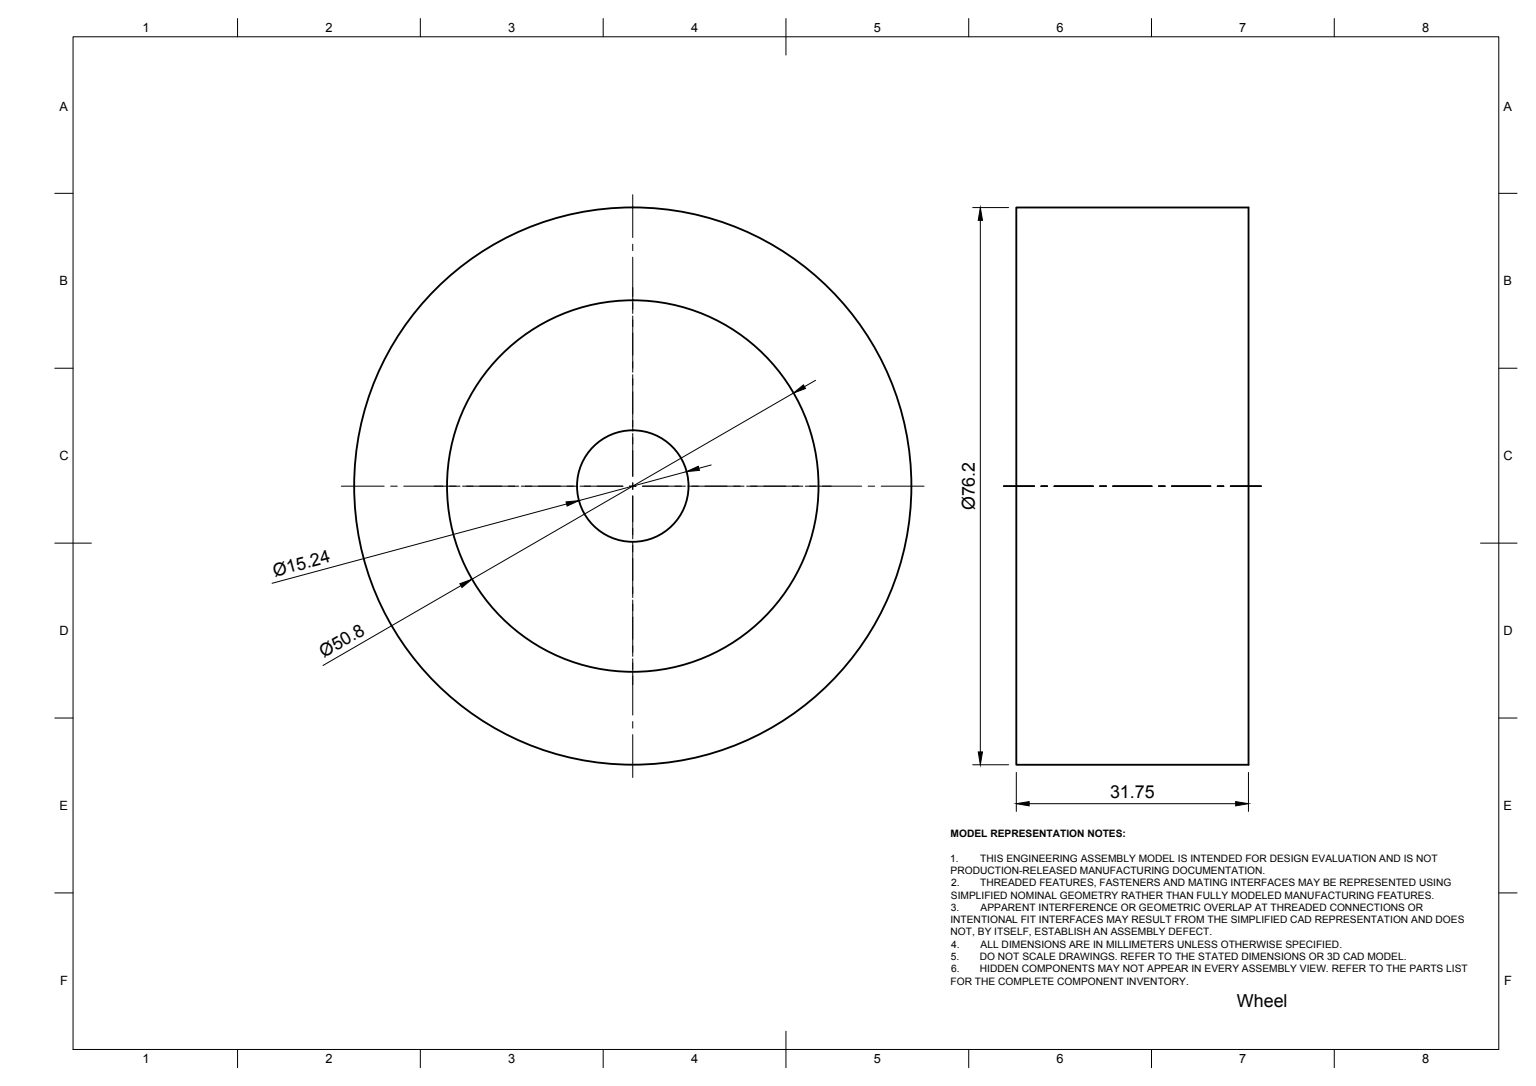
ISO-10303-21;
HEADER;
/* Generated by software containing ST-Developer
 * from STEP Tools, Inc. (www.steptools.com) 
 */

FILE_DESCRIPTION(
/* description */ ('Wheel Holder-Mirrored'),
/* implementation_level */ '2;1');

FILE_NAME(
/* name */ 'Wheel.step',
/* time_stamp */ '2026-10-07T09:01:46-07:00',
/* author */ (''),
/* organization */ (''),
/* preprocessor_version */ 'ST-DEVELOPER v20.2',
/* originating_system */ 'Autodesk Translation Framework v15.15.0.0',
/* authorisation */ '');

FILE_SCHEMA (('AUTOMOTIVE_DESIGN { 1 0 10303 214 3 1 1 }'));
ENDSEC;

DATA;
#10=MECHANICAL_DESIGN_GEOMETRIC_PRESENTATION_REPRESENTATION('',(#198),#3832);
#186=SHAPE_REPRESENTATION_RELATIONSHIP('SRR','None',#3863,#192);
#192=ADVANCED_BREP_SHAPE_REPRESENTATION('',(#204),#3826);
#198=STYLED_ITEM('',(#3902),#204);
#204=MANIFOLD_SOLID_BREP('Body1',#1783);
#210=FACE_BOUND('',#381,.T.);
#211=FACE_BOUND('',#383,.T.);
#212=FACE_BOUND('',#386,.T.);
#213=FACE_BOUND('',#388,.T.);
#227=PLANE('',#1867);
#228=PLANE('',#1868);
#229=PLANE('',#1872);
#230=PLANE('',#1873);
#273=FACE_OUTER_BOUND('',#377,.T.);
#274=FACE_OUTER_BOUND('',#378,.T.);
#275=FACE_OUTER_BOUND('',#379,.T.);
#276=FACE_OUTER_BOUND('',#380,.T.);
#277=FACE_OUTER_BOUND('',#382,.T.);
#278=FACE_OUTER_BOUND('',#384,.T.);
#279=FACE_OUTER_BOUND('',#385,.T.);
#280=FACE_OUTER_BOUND('',#387,.T.);
#377=EDGE_LOOP('',(#1153,#1154,#1155,#1156));
#378=EDGE_LOOP('',(#1157,#1158,#1159,#1160));
#379=EDGE_LOOP('',(#1161,#1162,#1163,#1164));
#380=EDGE_LOOP('',(#1165));
#381=EDGE_LOOP('',(#1166));
#382=EDGE_LOOP('',(#1167));
#383=EDGE_LOOP('',(#1168));
#384=EDGE_LOOP('',(#1169,#1170,#1171,#1172));
#385=EDGE_LOOP('',(#1173));
#386=EDGE_LOOP('',(#1174));
#387=EDGE_LOOP('',(#1175));
#388=EDGE_LOOP('',(#1176));
#498=LINE('',#2531,#591);
#499=LINE('',#2537,#592);
#500=LINE('',#2543,#593);
#501=LINE('',#2551,#594);
#591=VECTOR('',#2056,0.0254);
#592=VECTOR('',#2063,0.0254);
#593=VECTOR('',#2070,0.0381);
#594=VECTOR('',#2081,0.00762);
#684=CIRCLE('',#1859,0.0254);
#685=CIRCLE('',#1860,0.0254);
#686=CIRCLE('',#1862,0.0254);
#687=CIRCLE('',#1863,0.0254);
#688=CIRCLE('',#1865,0.0381);
#689=CIRCLE('',#1866,0.0381);
#690=CIRCLE('',#1870,0.00762);
#691=CIRCLE('',#1871,0.00762);
#746=VERTEX_POINT('',#2528);
#747=VERTEX_POINT('',#2530);
#748=VERTEX_POINT('',#2534);
#749=VERTEX_POINT('',#2536);
#750=VERTEX_POINT('',#2540);
#751=VERTEX_POINT('',#2542);
#752=VERTEX_POINT('',#2548);
#753=VERTEX_POINT('',#2550);
#903=EDGE_CURVE('',#746,#746,#684,.T.);
#904=EDGE_CURVE('',#746,#747,#498,.T.);
#905=EDGE_CURVE('',#747,#747,#685,.T.);
#906=EDGE_CURVE('',#748,#748,#686,.T.);
#907=EDGE_CURVE('',#748,#749,#499,.T.);
#908=EDGE_CURVE('',#749,#749,#687,.T.);
#909=EDGE_CURVE('',#750,#750,#688,.T.);
#910=EDGE_CURVE('',#750,#751,#500,.T.);
#911=EDGE_CURVE('',#751,#751,#689,.T.);
#912=EDGE_CURVE('',#752,#752,#690,.T.);
#913=EDGE_CURVE('',#752,#753,#501,.T.);
#914=EDGE_CURVE('',#753,#753,#691,.T.);
#1153=ORIENTED_EDGE('',*,*,#903,.T.);
#1154=ORIENTED_EDGE('',*,*,#904,.T.);
#1155=ORIENTED_EDGE('',*,*,#905,.F.);
#1156=ORIENTED_EDGE('',*,*,#904,.F.);
#1157=ORIENTED_EDGE('',*,*,#906,.T.);
#1158=ORIENTED_EDGE('',*,*,#907,.T.);
#1159=ORIENTED_EDGE('',*,*,#908,.F.);
#1160=ORIENTED_EDGE('',*,*,#907,.F.);
#1161=ORIENTED_EDGE('',*,*,#909,.T.);
#1162=ORIENTED_EDGE('',*,*,#910,.T.);
#1163=ORIENTED_EDGE('',*,*,#911,.F.);
#1164=ORIENTED_EDGE('',*,*,#910,.F.);
#1165=ORIENTED_EDGE('',*,*,#911,.T.);
#1166=ORIENTED_EDGE('',*,*,#906,.F.);
#1167=ORIENTED_EDGE('',*,*,#909,.F.);
#1168=ORIENTED_EDGE('',*,*,#905,.T.);
#1169=ORIENTED_EDGE('',*,*,#912,.T.);
#1170=ORIENTED_EDGE('',*,*,#913,.T.);
#1171=ORIENTED_EDGE('',*,*,#914,.F.);
#1172=ORIENTED_EDGE('',*,*,#913,.F.);
#1173=ORIENTED_EDGE('',*,*,#908,.T.);
#1174=ORIENTED_EDGE('',*,*,#912,.F.);
#1175=ORIENTED_EDGE('',*,*,#903,.F.);
#1176=ORIENTED_EDGE('',*,*,#914,.T.);
#1653=CYLINDRICAL_SURFACE('',#1858,0.0254);
#1654=CYLINDRICAL_SURFACE('',#1861,0.0254);
#1655=CYLINDRICAL_SURFACE('',#1864,0.0381);
#1656=CYLINDRICAL_SURFACE('',#1869,0.00762);
#1679=ADVANCED_FACE('',(#273),#1653,.F.);
#1680=ADVANCED_FACE('',(#274),#1654,.F.);
#1681=ADVANCED_FACE('',(#275),#1655,.T.);
#1682=ADVANCED_FACE('',(#276,#210),#227,.T.);
#1683=ADVANCED_FACE('',(#277,#211),#228,.F.);
#1684=ADVANCED_FACE('',(#278),#1656,.F.);
#1685=ADVANCED_FACE('',(#279,#212),#229,.T.);
#1686=ADVANCED_FACE('',(#280,#213),#230,.F.);
#1783=CLOSED_SHELL('',(#1679,#1680,#1681,#1682,#1683,#1684,#1685,#1686));
#1857=AXIS2_PLACEMENT_3D('',#2526,#2050,#2051);
#1858=AXIS2_PLACEMENT_3D('',#2527,#2052,#2053);
#1859=AXIS2_PLACEMENT_3D('',#2529,#2054,#2055);
#1860=AXIS2_PLACEMENT_3D('',#2532,#2057,#2058);
#1861=AXIS2_PLACEMENT_3D('',#2533,#2059,#2060);
#1862=AXIS2_PLACEMENT_3D('',#2535,#2061,#2062);
#1863=AXIS2_PLACEMENT_3D('',#2538,#2064,#2065);
#1864=AXIS2_PLACEMENT_3D('',#2539,#2066,#2067);
#1865=AXIS2_PLACEMENT_3D('',#2541,#2068,#2069);
#1866=AXIS2_PLACEMENT_3D('',#2544,#2071,#2072);
#1867=AXIS2_PLACEMENT_3D('',#2545,#2073,#2074);
#1868=AXIS2_PLACEMENT_3D('',#2546,#2075,#2076);
#1869=AXIS2_PLACEMENT_3D('',#2547,#2077,#2078);
#1870=AXIS2_PLACEMENT_3D('',#2549,#2079,#2080);
#1871=AXIS2_PLACEMENT_3D('',#2552,#2082,#2083);
#1872=AXIS2_PLACEMENT_3D('',#2553,#2084,#2085);
#1873=AXIS2_PLACEMENT_3D('',#2554,#2086,#2087);
#2050=DIRECTION('axis',(0.,0.,1.));
#2051=DIRECTION('refdir',(1.,0.,0.));
#2052=DIRECTION('center_axis',(-1.,0.,0.));
#2053=DIRECTION('ref_axis',(0.,0.,1.));
#2054=DIRECTION('center_axis',(1.,0.,0.));
#2055=DIRECTION('ref_axis',(0.,0.,-1.));
#2056=DIRECTION('',(-1.,0.,0.));
#2057=DIRECTION('center_axis',(1.,0.,0.));
#2058=DIRECTION('ref_axis',(0.,0.,-1.));
#2059=DIRECTION('center_axis',(-1.,0.,0.));
#2060=DIRECTION('ref_axis',(0.,0.,1.));
#2061=DIRECTION('center_axis',(1.,0.,0.));
#2062=DIRECTION('ref_axis',(0.,0.,-1.));
#2063=DIRECTION('',(-1.,0.,0.));
#2064=DIRECTION('center_axis',(1.,0.,0.));
#2065=DIRECTION('ref_axis',(0.,0.,-1.));
#2066=DIRECTION('center_axis',(-1.,0.,0.));
#2067=DIRECTION('ref_axis',(0.,0.,1.));
#2068=DIRECTION('center_axis',(1.,0.,0.));
#2069=DIRECTION('ref_axis',(0.,0.,-1.));
#2070=DIRECTION('',(1.,0.,0.));
#2071=DIRECTION('center_axis',(1.,0.,0.));
#2072=DIRECTION('ref_axis',(0.,0.,-1.));
#2073=DIRECTION('center_axis',(1.,0.,0.));
#2074=DIRECTION('ref_axis',(0.,1.,0.));
#2075=DIRECTION('center_axis',(1.,0.,0.));
#2076=DIRECTION('ref_axis',(0.,1.,0.));
#2077=DIRECTION('center_axis',(-1.,0.,0.));
#2078=DIRECTION('ref_axis',(0.,0.,1.));
#2079=DIRECTION('center_axis',(1.,0.,0.));
#2080=DIRECTION('ref_axis',(0.,0.,-1.));
#2081=DIRECTION('',(-1.,0.,0.));
#2082=DIRECTION('center_axis',(1.,0.,0.));
#2083=DIRECTION('ref_axis',(0.,0.,-1.));
#2084=DIRECTION('center_axis',(1.,0.,0.));
#2085=DIRECTION('ref_axis',(0.,1.,0.));
#2086=DIRECTION('center_axis',(1.,0.,0.));
#2087=DIRECTION('ref_axis',(0.,1.,0.));
#2526=CARTESIAN_POINT('',(0.,0.,0.));
#2527=CARTESIAN_POINT('Origin',(0.015875,0.,1.55530143491714E-18));
#2528=CARTESIAN_POINT('',(-0.01143,0.,-0.0254));
#2529=CARTESIAN_POINT('Origin',(-0.01143,0.,1.55530143491714E-18));
#2530=CARTESIAN_POINT('',(-0.015875,0.,-0.0254));
#2531=CARTESIAN_POINT('',(0.015875,-3.11060286983428E-18,-0.0254));
#2532=CARTESIAN_POINT('Origin',(-0.015875,0.,1.55530143491714E-18));
#2533=CARTESIAN_POINT('Origin',(0.015875,0.,1.55530143491714E-18));
#2534=CARTESIAN_POINT('',(0.015875,0.,-0.0254));
#2535=CARTESIAN_POINT('Origin',(0.015875,0.,1.55530143491714E-18));
#2536=CARTESIAN_POINT('',(0.01143,0.,-0.0254));
#2537=CARTESIAN_POINT('',(0.015875,-3.11060286983428E-18,-0.0254));
#2538=CARTESIAN_POINT('Origin',(0.01143,0.,1.55530143491714E-18));
#2539=CARTESIAN_POINT('Origin',(0.015875,0.,2.33295215237571E-18));
#2540=CARTESIAN_POINT('',(-0.015875,0.,-0.0381));
#2541=CARTESIAN_POINT('Origin',(-0.015875,0.,2.33295215237571E-18));
#2542=CARTESIAN_POINT('',(0.015875,0.,-0.0381));
#2543=CARTESIAN_POINT('',(0.015875,-4.66590430475142E-18,-0.0381));
#2544=CARTESIAN_POINT('Origin',(0.015875,0.,2.33295215237571E-18));
#2545=CARTESIAN_POINT('Origin',(0.015875,0.,0.));
#2546=CARTESIAN_POINT('Origin',(-0.015875,0.,0.));
#2547=CARTESIAN_POINT('Origin',(0.01143,0.,4.66590430475142E-19));
#2548=CARTESIAN_POINT('',(0.01143,0.,-0.00762));
#2549=CARTESIAN_POINT('Origin',(0.01143,0.,4.66590430475142E-19));
#2550=CARTESIAN_POINT('',(-0.01143,0.,-0.00762));
#2551=CARTESIAN_POINT('',(0.01143,-9.33180860950283E-19,-0.00762));
#2552=CARTESIAN_POINT('Origin',(-0.01143,0.,4.66590430475142E-19));
#2553=CARTESIAN_POINT('Origin',(0.01143,0.,0.));
#2554=CARTESIAN_POINT('Origin',(-0.01143,0.,0.));
#3818=UNCERTAINTY_MEASURE_WITH_UNIT(LENGTH_MEASURE(1.E-5),#3833,
'DISTANCE_ACCURACY_VALUE',
'Maximum model space distance between geometric entities at asserted c
onnectivities');
#3824=UNCERTAINTY_MEASURE_WITH_UNIT(LENGTH_MEASURE(1.E-5),#3833,
'DISTANCE_ACCURACY_VALUE',
'Maximum model space distance between geometric entities at asserted c
onnectivities');
#3826=(
GEOMETRIC_REPRESENTATION_CONTEXT(3)
GLOBAL_UNCERTAINTY_ASSIGNED_CONTEXT((#3818))
GLOBAL_UNIT_ASSIGNED_CONTEXT((#3833,#3834,#3835))
REPRESENTATION_CONTEXT('','3D')
);
#3832=(
GEOMETRIC_REPRESENTATION_CONTEXT(3)
GLOBAL_UNCERTAINTY_ASSIGNED_CONTEXT((#3824))
GLOBAL_UNIT_ASSIGNED_CONTEXT((#3833,#3834,#3835))
REPRESENTATION_CONTEXT('','3D')
);
#3833=(
LENGTH_UNIT()
NAMED_UNIT(*)
SI_UNIT($,.METRE.)
);
#3834=(
NAMED_UNIT(*)
PLANE_ANGLE_UNIT()
SI_UNIT($,.RADIAN.)
);
#3835=(
NAMED_UNIT(*)
SI_UNIT($,.STERADIAN.)
SOLID_ANGLE_UNIT()
);
#3837=SHAPE_DEFINITION_REPRESENTATION(#3844,#3863);
#3844=PRODUCT_DEFINITION_SHAPE('',$,#3871);
#3863=SHAPE_REPRESENTATION('',(#1857),#3826);
#3869=PRODUCT_DEFINITION_CONTEXT('part definition',#3892,'design');
#3871=PRODUCT_DEFINITION('2026-10-07-15-35-32-214','Wheel',#3878,#3869);
#3878=PRODUCT_DEFINITION_FORMATION('',$,#3895);
#3892=APPLICATION_CONTEXT(
'Core Data for Automotive Mechanical Design Process');
#3893=PRODUCT_CONTEXT('part definition',#3892,'mechanical');
#3895=PRODUCT('2026-10-07-15-35-32-214','Wheel','Wheel',(#3893));
#3902=PRESENTATION_STYLE_ASSIGNMENT((#3908));
#3908=SURFACE_STYLE_USAGE(.BOTH.,#3914);
#3914=SURFACE_SIDE_STYLE('',(#3920));
#3920=SURFACE_STYLE_FILL_AREA(#3926);
#3926=FILL_AREA_STYLE('Opaque(59,97,180)',(#3932));
#3932=FILL_AREA_STYLE_COLOUR('Opaque(59,97,180)',#3938);
#3938=COLOUR_RGB('Opaque(59,97,180)', 0.09019608, 0.27058824, 0.51372549);
ENDSEC;
END-ISO-10303-21;
